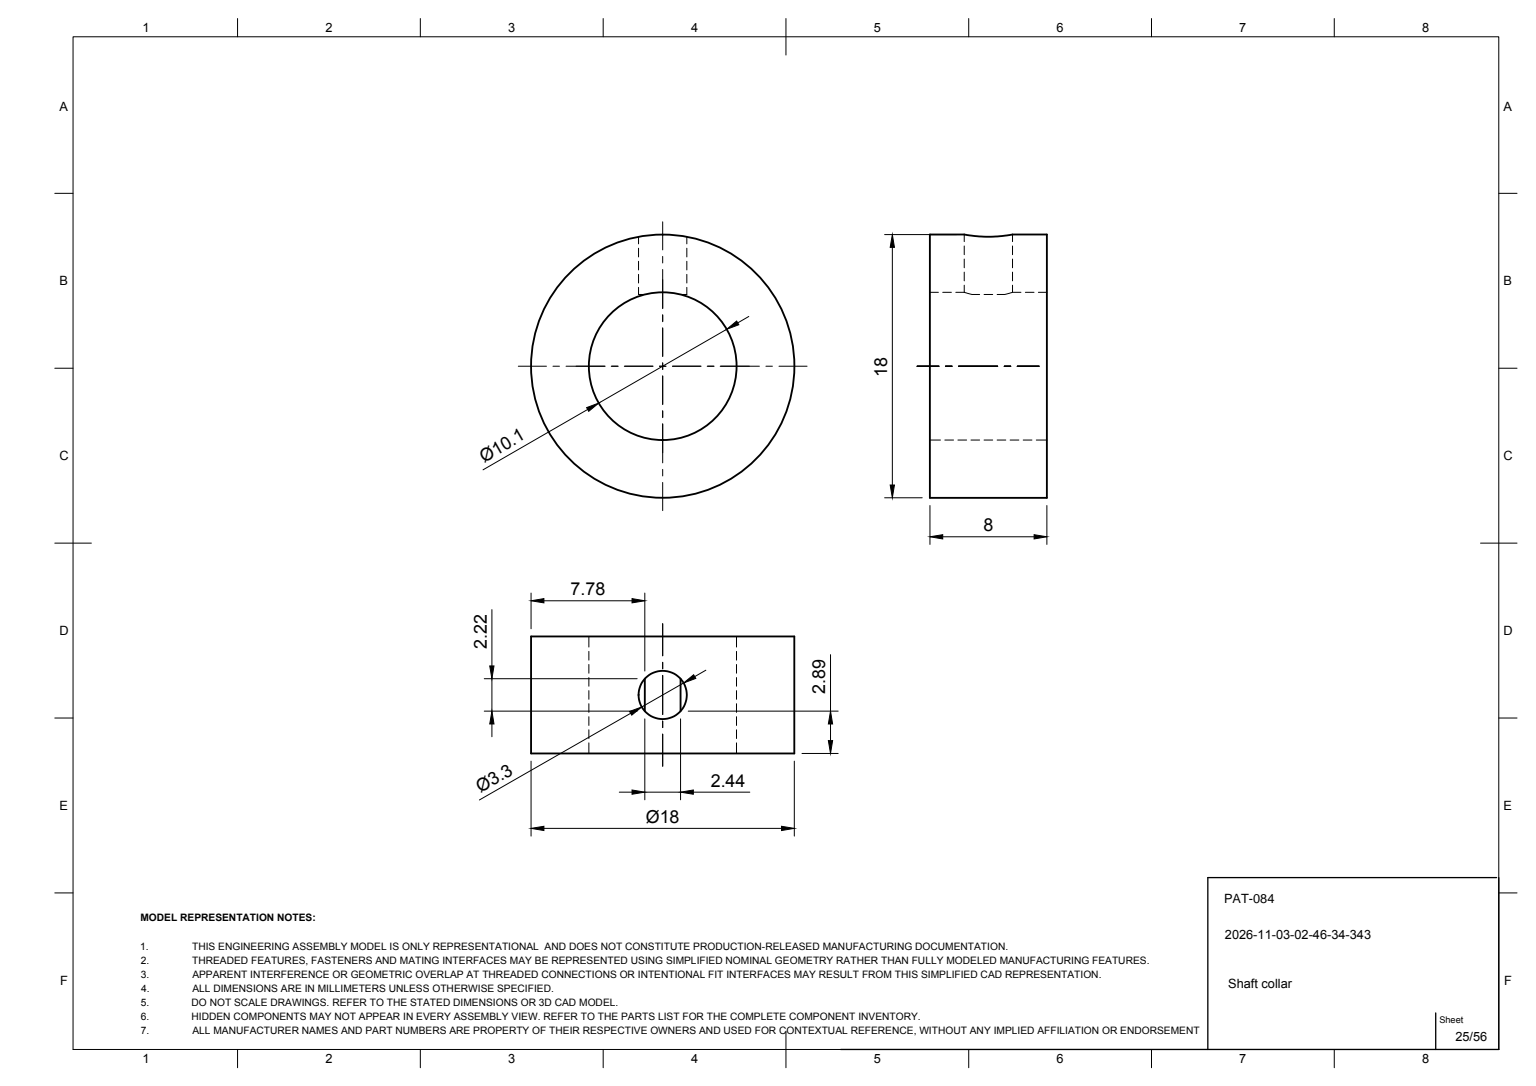
ISO-10303-21;
HEADER;
/* Generated by software containing ST-Developer
 * from STEP Tools, Inc. (www.steptools.com) 
 */

FILE_DESCRIPTION(
/* description */ ('Quick-return (Whitworth) mechanism'),
/* implementation_level */ '2;1');

FILE_NAME(
/* name */ 'Shaft collar.step',
/* time_stamp */ '2026-10-28T03:25:57-07:00',
/* author */ (''),
/* organization */ (''),
/* preprocessor_version */ 'ST-DEVELOPER v20.2',
/* originating_system */ 'Autodesk Translation Framework v15.17.0.0',
/* authorisation */ '');

FILE_SCHEMA (('AUTOMOTIVE_DESIGN { 1 0 10303 214 3 1 1 }'));
ENDSEC;

DATA;
#10=MECHANICAL_DESIGN_GEOMETRIC_PRESENTATION_REPRESENTATION('',(#514),#14878);
#392=B_SPLINE_CURVE_WITH_KNOTS('',3,(#13493,#13494,#13495,#13496,#13497,
#13498,#13499,#13500,#13501,#13502,#13503,#13504,#13505,#13506),
 .UNSPECIFIED.,.F.,.F.,(4,2,2,2,2,2,4),(0.618551524396291,0.626563103102765,
0.689203386094988,0.751843669087211,0.814483952079434,0.877124235071657,
0.88513581377813),.UNSPECIFIED.);
#393=B_SPLINE_CURVE_WITH_KNOTS('',3,(#13510,#13511,#13512,#13513,#13514,
#13515,#13516,#13517),.UNSPECIFIED.,.F.,.F.,(4,2,2,4),(0.250614556362404,
0.313254839354627,0.37589512234685,0.383906701053323),.UNSPECIFIED.);
#394=B_SPLINE_CURVE_WITH_KNOTS('',3,(#13521,#13522,#13523,#13524,#13525,
#13526,#13527,#13528,#13529,#13530,#13531,#13532,#13533,#13534,#13535,#13536,
#13537,#13538,#13539,#13540,#13541,#13542,#13543,#13544,#13545,#13546),
 .UNSPECIFIED.,.F.,.F.,(4,2,2,2,2,2,2,2,2,2,2,2,4),(0.,0.0623062782223143,
0.124612556444629,0.186916384615149,0.249220212785669,0.31152404095619,
0.37382786912671,0.436134147349024,0.498440425571339,0.560746703793653,
0.623052982015967,0.685356810186488,0.747660638357008),.UNSPECIFIED.);
#395=B_SPLINE_CURVE_WITH_KNOTS('',3,(#13547,#13548,#13549,#13550,#13551,
#13552,#13553,#13554,#13555,#13556),.UNSPECIFIED.,.F.,.F.,(4,2,2,2,4),(0.747660638357008,
0.809964466527529,0.872268294698049,0.934574572920363,0.996880851142677),
 .UNSPECIFIED.);
#396=B_SPLINE_CURVE_WITH_KNOTS('',3,(#13557,#13558,#13559,#13560,#13561,
#13562,#13563,#13564),.UNSPECIFIED.,.F.,.F.,(4,2,2,4),(0.117322411671485,
0.125333990377958,0.187974273370181,0.250614556362404),.UNSPECIFIED.);
#418=SHAPE_REPRESENTATION_RELATIONSHIP('SRR','None',#15088,#462);
#462=ADVANCED_BREP_SHAPE_REPRESENTATION('',(#566),#14845);
#514=STYLED_ITEM('',(#15406),#566);
#566=MANIFOLD_SOLID_BREP('Body1',#7868);
#711=FACE_BOUND('',#1863,.T.);
#712=FACE_BOUND('',#1865,.T.);
#713=FACE_BOUND('',#1867,.T.);
#714=FACE_BOUND('',#1869,.T.);
#886=PLANE('',#8896);
#887=PLANE('',#8900);
#888=PLANE('',#8907);
#889=PLANE('',#8908);
#1273=FACE_OUTER_BOUND('',#1859,.T.);
#1274=FACE_OUTER_BOUND('',#1860,.T.);
#1275=FACE_OUTER_BOUND('',#1861,.T.);
#1276=FACE_OUTER_BOUND('',#1862,.T.);
#1277=FACE_OUTER_BOUND('',#1864,.T.);
#1278=FACE_OUTER_BOUND('',#1866,.T.);
#1279=FACE_OUTER_BOUND('',#1868,.T.);
#1859=EDGE_LOOP('',(#6226,#6227));
#1860=EDGE_LOOP('',(#6228,#6229,#6230,#6231,#6232,#6233,#6234,#6235,#6236));
#1861=EDGE_LOOP('',(#6237,#6238));
#1862=EDGE_LOOP('',(#6239,#6240,#6241,#6242));
#1863=EDGE_LOOP('',(#6243,#6244,#6245,#6246,#6247));
#1864=EDGE_LOOP('',(#6248,#6249,#6250,#6251));
#1865=EDGE_LOOP('',(#6252,#6253));
#1866=EDGE_LOOP('',(#6254));
#1867=EDGE_LOOP('',(#6255));
#1868=EDGE_LOOP('',(#6256));
#1869=EDGE_LOOP('',(#6257));
#2366=LINE('',#13489,#2889);
#2367=LINE('',#13519,#2890);
#2368=LINE('',#13566,#2891);
#2369=LINE('',#13571,#2892);
#2370=LINE('',#13577,#2893);
#2889=VECTOR('',#10619,1.);
#2890=VECTOR('',#10626,0.165);
#2891=VECTOR('',#10629,1.);
#2892=VECTOR('',#10634,0.505);
#2893=VECTOR('',#10641,0.9);
#3476=CIRCLE('',#8897,0.165);
#3477=CIRCLE('',#8899,0.165);
#3478=CIRCLE('',#8902,0.505);
#3479=CIRCLE('',#8903,0.505);
#3480=CIRCLE('',#8905,0.9);
#3481=CIRCLE('',#8906,0.9);
#3963=VERTEX_POINT('',#13487);
#3964=VERTEX_POINT('',#13488);
#3965=VERTEX_POINT('',#13492);
#3966=VERTEX_POINT('',#13507);
#3967=VERTEX_POINT('',#13509);
#3968=VERTEX_POINT('',#13518);
#3969=VERTEX_POINT('',#13520);
#3970=VERTEX_POINT('',#13568);
#3971=VERTEX_POINT('',#13570);
#3972=VERTEX_POINT('',#13574);
#3973=VERTEX_POINT('',#13576);
#4770=EDGE_CURVE('',#3963,#3964,#2366,.T.);
#4771=EDGE_CURVE('',#3963,#3964,#3476,.T.);
#4772=EDGE_CURVE('',#3965,#3963,#392,.T.);
#4773=EDGE_CURVE('',#3966,#3965,#3477,.T.);
#4774=EDGE_CURVE('',#3967,#3966,#393,.T.);
#4775=EDGE_CURVE('',#3967,#3968,#2367,.T.);
#4776=EDGE_CURVE('',#3969,#3968,#394,.T.);
#4777=EDGE_CURVE('',#3968,#3969,#395,.T.);
#4778=EDGE_CURVE('',#3964,#3967,#396,.T.);
#4779=EDGE_CURVE('',#3966,#3965,#2368,.T.);
#4780=EDGE_CURVE('',#3970,#3970,#3478,.T.);
#4781=EDGE_CURVE('',#3970,#3971,#2369,.T.);
#4782=EDGE_CURVE('',#3971,#3971,#3479,.T.);
#4783=EDGE_CURVE('',#3972,#3972,#3480,.T.);
#4784=EDGE_CURVE('',#3972,#3973,#2370,.T.);
#4785=EDGE_CURVE('',#3973,#3973,#3481,.T.);
#6226=ORIENTED_EDGE('',*,*,#4770,.F.);
#6227=ORIENTED_EDGE('',*,*,#4771,.T.);
#6228=ORIENTED_EDGE('',*,*,#4772,.F.);
#6229=ORIENTED_EDGE('',*,*,#4773,.F.);
#6230=ORIENTED_EDGE('',*,*,#4774,.F.);
#6231=ORIENTED_EDGE('',*,*,#4775,.T.);
#6232=ORIENTED_EDGE('',*,*,#4776,.F.);
#6233=ORIENTED_EDGE('',*,*,#4777,.F.);
#6234=ORIENTED_EDGE('',*,*,#4775,.F.);
#6235=ORIENTED_EDGE('',*,*,#4778,.F.);
#6236=ORIENTED_EDGE('',*,*,#4771,.F.);
#6237=ORIENTED_EDGE('',*,*,#4779,.F.);
#6238=ORIENTED_EDGE('',*,*,#4773,.T.);
#6239=ORIENTED_EDGE('',*,*,#4780,.F.);
#6240=ORIENTED_EDGE('',*,*,#4781,.T.);
#6241=ORIENTED_EDGE('',*,*,#4782,.T.);
#6242=ORIENTED_EDGE('',*,*,#4781,.F.);
#6243=ORIENTED_EDGE('',*,*,#4778,.T.);
#6244=ORIENTED_EDGE('',*,*,#4774,.T.);
#6245=ORIENTED_EDGE('',*,*,#4779,.T.);
#6246=ORIENTED_EDGE('',*,*,#4772,.T.);
#6247=ORIENTED_EDGE('',*,*,#4770,.T.);
#6248=ORIENTED_EDGE('',*,*,#4783,.F.);
#6249=ORIENTED_EDGE('',*,*,#4784,.T.);
#6250=ORIENTED_EDGE('',*,*,#4785,.T.);
#6251=ORIENTED_EDGE('',*,*,#4784,.F.);
#6252=ORIENTED_EDGE('',*,*,#4776,.T.);
#6253=ORIENTED_EDGE('',*,*,#4777,.T.);
#6254=ORIENTED_EDGE('',*,*,#4783,.T.);
#6255=ORIENTED_EDGE('',*,*,#4780,.T.);
#6256=ORIENTED_EDGE('',*,*,#4785,.F.);
#6257=ORIENTED_EDGE('',*,*,#4782,.F.);
#7310=CYLINDRICAL_SURFACE('',#8898,0.165);
#7311=CYLINDRICAL_SURFACE('',#8901,0.505);
#7312=CYLINDRICAL_SURFACE('',#8904,0.9);
#7604=ADVANCED_FACE('',(#1273),#886,.T.);
#7605=ADVANCED_FACE('',(#1274),#7310,.F.);
#7606=ADVANCED_FACE('',(#1275),#887,.T.);
#7607=ADVANCED_FACE('',(#1276,#711),#7311,.F.);
#7608=ADVANCED_FACE('',(#1277,#712),#7312,.T.);
#7609=ADVANCED_FACE('',(#1278,#713),#888,.T.);
#7610=ADVANCED_FACE('',(#1279,#714),#889,.F.);
#7868=CLOSED_SHELL('',(#7604,#7605,#7606,#7607,#7608,#7609,#7610));
#8895=AXIS2_PLACEMENT_3D('',#13485,#10615,#10616);
#8896=AXIS2_PLACEMENT_3D('',#13486,#10617,#10618);
#8897=AXIS2_PLACEMENT_3D('',#13490,#10620,#10621);
#8898=AXIS2_PLACEMENT_3D('',#13491,#10622,#10623);
#8899=AXIS2_PLACEMENT_3D('',#13508,#10624,#10625);
#8900=AXIS2_PLACEMENT_3D('',#13565,#10627,#10628);
#8901=AXIS2_PLACEMENT_3D('',#13567,#10630,#10631);
#8902=AXIS2_PLACEMENT_3D('',#13569,#10632,#10633);
#8903=AXIS2_PLACEMENT_3D('',#13572,#10635,#10636);
#8904=AXIS2_PLACEMENT_3D('',#13573,#10637,#10638);
#8905=AXIS2_PLACEMENT_3D('',#13575,#10639,#10640);
#8906=AXIS2_PLACEMENT_3D('',#13578,#10642,#10643);
#8907=AXIS2_PLACEMENT_3D('',#13579,#10644,#10645);
#8908=AXIS2_PLACEMENT_3D('',#13580,#10646,#10647);
#10615=DIRECTION('axis',(0.,0.,1.));
#10616=DIRECTION('refdir',(1.,0.,0.));
#10617=DIRECTION('center_axis',(1.,0.,0.));
#10618=DIRECTION('ref_axis',(0.,0.,-1.));
#10619=DIRECTION('',(0.,0.,1.));
#10620=DIRECTION('center_axis',(1.,0.,0.));
#10621=DIRECTION('ref_axis',(0.,0.,-1.));
#10622=DIRECTION('center_axis',(1.,0.,0.));
#10623=DIRECTION('ref_axis',(0.,0.,-1.));
#10624=DIRECTION('center_axis',(1.,0.,0.));
#10625=DIRECTION('ref_axis',(0.,0.,-1.));
#10626=DIRECTION('',(1.,0.,0.));
#10627=DIRECTION('center_axis',(1.,0.,0.));
#10628=DIRECTION('ref_axis',(0.,0.,-1.));
#10629=DIRECTION('',(0.,0.,-1.));
#10630=DIRECTION('center_axis',(0.,0.,1.));
#10631=DIRECTION('ref_axis',(1.,0.,0.));
#10632=DIRECTION('center_axis',(0.,0.,-1.));
#10633=DIRECTION('ref_axis',(1.,0.,0.));
#10634=DIRECTION('',(0.,0.,-1.));
#10635=DIRECTION('center_axis',(0.,0.,-1.));
#10636=DIRECTION('ref_axis',(1.,0.,0.));
#10637=DIRECTION('center_axis',(0.,0.,1.));
#10638=DIRECTION('ref_axis',(1.,0.,0.));
#10639=DIRECTION('center_axis',(0.,0.,1.));
#10640=DIRECTION('ref_axis',(1.,0.,0.));
#10641=DIRECTION('',(0.,0.,-1.));
#10642=DIRECTION('center_axis',(0.,0.,1.));
#10643=DIRECTION('ref_axis',(1.,0.,0.));
#10644=DIRECTION('center_axis',(0.,0.,1.));
#10645=DIRECTION('ref_axis',(1.,0.,0.));
#10646=DIRECTION('center_axis',(0.,0.,1.));
#10647=DIRECTION('ref_axis',(1.,0.,0.));
#13485=CARTESIAN_POINT('',(0.,0.,0.));
#13486=CARTESIAN_POINT('Origin',(0.49,6.,1.4));
#13487=CARTESIAN_POINT('',(0.49,6.12216791722871,1.28909463493591));
#13488=CARTESIAN_POINT('',(0.49,6.12216791722871,1.51090536506409));
#13489=CARTESIAN_POINT('',(0.49,6.12216791722871,1.));
#13490=CARTESIAN_POINT('Origin',(0.49,6.,1.4));
#13491=CARTESIAN_POINT('Origin',(0.49,6.,1.4));
#13492=CARTESIAN_POINT('',(0.49,5.87783208277129,1.28909463493591));
#13493=CARTESIAN_POINT('Ctrl Pts',(0.49,5.87783208277129,1.28909463493591));
#13494=CARTESIAN_POINT('Ctrl Pts',(0.490448531679987,5.8796310863737,1.28711294069536));
#13495=CARTESIAN_POINT('Ctrl Pts',(0.490895245371684,5.88146510343477,1.28518965877367));
#13496=CARTESIAN_POINT('Ctrl Pts',(0.494795015531646,5.89788800698064,1.2687667552278));
#13497=CARTESIAN_POINT('Ctrl Pts',(0.498442514607594,5.91634028497757,1.25609154388858));
#13498=CARTESIAN_POINT('Ctrl Pts',(0.50357781976106,5.95695040395284,1.23920409039234));
#13499=CARTESIAN_POINT('Ctrl Pts',(0.505,5.97911990566926,1.235));
#13500=CARTESIAN_POINT('Ctrl Pts',(0.505,6.02088009433074,1.235));
#13501=CARTESIAN_POINT('Ctrl Pts',(0.50357781976106,6.04304959604716,1.23920409039234));
#13502=CARTESIAN_POINT('Ctrl Pts',(0.498442514607594,6.08365971502243,1.25609154388858));
#13503=CARTESIAN_POINT('Ctrl Pts',(0.494795015531646,6.10211199301936,1.2687667552278));
#13504=CARTESIAN_POINT('Ctrl Pts',(0.490895245371684,6.11853489656523,1.28518965877367));
#13505=CARTESIAN_POINT('Ctrl Pts',(0.490448531679987,6.1203689136263,1.28711294069536));
#13506=CARTESIAN_POINT('Ctrl Pts',(0.49,6.12216791722871,1.28909463493591));
#13507=CARTESIAN_POINT('',(0.49,5.87783208277129,1.51090536506409));
#13508=CARTESIAN_POINT('Origin',(0.49,6.,1.4));
#13509=CARTESIAN_POINT('',(0.505,6.,1.565));
#13510=CARTESIAN_POINT('Ctrl Pts',(0.505,6.,1.565));
#13511=CARTESIAN_POINT('Ctrl Pts',(0.505,5.97911990566926,1.565));
#13512=CARTESIAN_POINT('Ctrl Pts',(0.50357781976106,5.95695040395284,1.56079590960766));
#13513=CARTESIAN_POINT('Ctrl Pts',(0.498442514607594,5.91634028497757,1.54390845611142));
#13514=CARTESIAN_POINT('Ctrl Pts',(0.494795015531646,5.89788800698064,1.5312332447722));
#13515=CARTESIAN_POINT('Ctrl Pts',(0.490895245371684,5.88146510343477,1.51481034122633));
#13516=CARTESIAN_POINT('Ctrl Pts',(0.490448531679987,5.8796310863737,1.51288705930464));
#13517=CARTESIAN_POINT('Ctrl Pts',(0.49,5.87783208277129,1.51090536506409));
#13518=CARTESIAN_POINT('',(0.9,6.,1.565));
#13519=CARTESIAN_POINT('',(0.49,6.,1.565));
#13520=CARTESIAN_POINT('',(0.884745726183518,6.165,1.4));
#13521=CARTESIAN_POINT('Ctrl Pts',(0.884745726183518,6.165,1.4));
#13522=CARTESIAN_POINT('Ctrl Pts',(0.884745726183518,6.165,1.37923124059256));
#13523=CARTESIAN_POINT('Ctrl Pts',(0.885552759505264,6.16083971900758,1.35711110492666));
#13524=CARTESIAN_POINT('Ctrl Pts',(0.888448648150043,6.14398647021669,1.31647293736623));
#13525=CARTESIAN_POINT('Ctrl Pts',(0.890493604851638,6.13129599381419,1.29795075602263));
#13526=CARTESIAN_POINT('Ctrl Pts',(0.89431723432394,6.10204981900812,1.26870458121656));
#13527=CARTESIAN_POINT('Ctrl Pts',(0.896347088899543,6.08352739209068,1.25601365401642));
#13528=CARTESIAN_POINT('Ctrl Pts',(0.899208271860583,6.04288837609341,1.23916007816136));
#13529=CARTESIAN_POINT('Ctrl Pts',(0.9,6.02076794272351,1.235));
#13530=CARTESIAN_POINT('Ctrl Pts',(0.9,5.97923205727649,1.235));
#13531=CARTESIAN_POINT('Ctrl Pts',(0.899208271860583,5.95711162390659,1.23916007816136));
#13532=CARTESIAN_POINT('Ctrl Pts',(0.896347088899543,5.91647260790932,1.25601365401642));
#13533=CARTESIAN_POINT('Ctrl Pts',(0.89431723432394,5.89795018099188,1.26870458121656));
#13534=CARTESIAN_POINT('Ctrl Pts',(0.890493604851638,5.86870400618581,1.29795075602263));
#13535=CARTESIAN_POINT('Ctrl Pts',(0.888448648150043,5.85601352978331,1.31647293736623));
#13536=CARTESIAN_POINT('Ctrl Pts',(0.885552759505264,5.83916028099242,1.35711110492666));
#13537=CARTESIAN_POINT('Ctrl Pts',(0.884745726183518,5.835,1.37923124059256));
#13538=CARTESIAN_POINT('Ctrl Pts',(0.884745726183518,5.835,1.42076875940744));
#13539=CARTESIAN_POINT('Ctrl Pts',(0.885552759505264,5.83916028099242,1.44288889507334));
#13540=CARTESIAN_POINT('Ctrl Pts',(0.888448648150043,5.85601352978331,1.48352706263377));
#13541=CARTESIAN_POINT('Ctrl Pts',(0.890493604851638,5.86870400618581,1.50204924397737));
#13542=CARTESIAN_POINT('Ctrl Pts',(0.89431723432394,5.89795018099188,1.53129541878344));
#13543=CARTESIAN_POINT('Ctrl Pts',(0.896347088899543,5.91647260790932,1.54398634598358));
#13544=CARTESIAN_POINT('Ctrl Pts',(0.899208271860583,5.95711162390659,1.56083992183864));
#13545=CARTESIAN_POINT('Ctrl Pts',(0.9,5.97923205727649,1.565));
#13546=CARTESIAN_POINT('Ctrl Pts',(0.9,6.,1.565));
#13547=CARTESIAN_POINT('Ctrl Pts',(0.9,6.,1.565));
#13548=CARTESIAN_POINT('Ctrl Pts',(0.9,6.02076794272351,1.565));
#13549=CARTESIAN_POINT('Ctrl Pts',(0.899208271860583,6.04288837609341,1.56083992183864));
#13550=CARTESIAN_POINT('Ctrl Pts',(0.896347088899543,6.08352739209068,1.54398634598358));
#13551=CARTESIAN_POINT('Ctrl Pts',(0.89431723432394,6.10204981900812,1.53129541878344));
#13552=CARTESIAN_POINT('Ctrl Pts',(0.890493604851638,6.13129599381419,1.50204924397737));
#13553=CARTESIAN_POINT('Ctrl Pts',(0.888448648150043,6.14398647021669,1.48352706263377));
#13554=CARTESIAN_POINT('Ctrl Pts',(0.885552759505264,6.16083971900758,1.44288889507334));
#13555=CARTESIAN_POINT('Ctrl Pts',(0.884745726183518,6.165,1.42076875940744));
#13556=CARTESIAN_POINT('Ctrl Pts',(0.884745726183518,6.165,1.4));
#13557=CARTESIAN_POINT('Ctrl Pts',(0.49,6.12216791722871,1.51090536506409));
#13558=CARTESIAN_POINT('Ctrl Pts',(0.490448531679987,6.1203689136263,1.51288705930464));
#13559=CARTESIAN_POINT('Ctrl Pts',(0.490895245371684,6.11853489656523,1.51481034122633));
#13560=CARTESIAN_POINT('Ctrl Pts',(0.494795015531646,6.10211199301936,1.5312332447722));
#13561=CARTESIAN_POINT('Ctrl Pts',(0.498442514607594,6.08365971502243,1.54390845611142));
#13562=CARTESIAN_POINT('Ctrl Pts',(0.50357781976106,6.04304959604716,1.56079590960766));
#13563=CARTESIAN_POINT('Ctrl Pts',(0.505,6.02088009433074,1.565));
#13564=CARTESIAN_POINT('Ctrl Pts',(0.505,6.,1.565));
#13565=CARTESIAN_POINT('Origin',(0.49,6.,1.4));
#13566=CARTESIAN_POINT('',(0.49,5.87783208277129,1.));
#13567=CARTESIAN_POINT('Origin',(0.,6.,1.));
#13568=CARTESIAN_POINT('',(-0.505,6.,1.8));
#13569=CARTESIAN_POINT('Origin',(0.,6.,1.8));
#13570=CARTESIAN_POINT('',(-0.505,6.,1.));
#13571=CARTESIAN_POINT('',(-0.505,6.,1.));
#13572=CARTESIAN_POINT('Origin',(0.,6.,1.));
#13573=CARTESIAN_POINT('Origin',(0.,6.,1.));
#13574=CARTESIAN_POINT('',(-0.9,6.,1.8));
#13575=CARTESIAN_POINT('Origin',(0.,6.,1.8));
#13576=CARTESIAN_POINT('',(-0.9,6.,1.));
#13577=CARTESIAN_POINT('',(-0.9,6.,1.));
#13578=CARTESIAN_POINT('Origin',(0.,6.,1.));
#13579=CARTESIAN_POINT('Origin',(0.,6.,1.8));
#13580=CARTESIAN_POINT('Origin',(0.,6.,1.));
#14791=UNCERTAINTY_MEASURE_WITH_UNIT(LENGTH_MEASURE(0.001),#14879,
'DISTANCE_ACCURACY_VALUE',
'Maximum model space distance between geometric entities at asserted c
onnectivities');
#14824=UNCERTAINTY_MEASURE_WITH_UNIT(LENGTH_MEASURE(0.001),#14879,
'DISTANCE_ACCURACY_VALUE',
'Maximum model space distance between geometric entities at asserted c
onnectivities');
#14845=(
GEOMETRIC_REPRESENTATION_CONTEXT(3)
GLOBAL_UNCERTAINTY_ASSIGNED_CONTEXT((#14791))
GLOBAL_UNIT_ASSIGNED_CONTEXT((#14879,#14881,#14882))
REPRESENTATION_CONTEXT('','3D')
);
#14878=(
GEOMETRIC_REPRESENTATION_CONTEXT(3)
GLOBAL_UNCERTAINTY_ASSIGNED_CONTEXT((#14824))
GLOBAL_UNIT_ASSIGNED_CONTEXT((#14879,#14881,#14882))
REPRESENTATION_CONTEXT('','3D')
);
#14879=(
LENGTH_UNIT()
NAMED_UNIT(*)
SI_UNIT(.CENTI.,.METRE.)
);
#14881=(
NAMED_UNIT(*)
PLANE_ANGLE_UNIT()
SI_UNIT($,.RADIAN.)
);
#14882=(
NAMED_UNIT(*)
SI_UNIT($,.STERADIAN.)
SOLID_ANGLE_UNIT()
);
#14903=SHAPE_DEFINITION_REPRESENTATION(#14961,#15088);
#14961=PRODUCT_DEFINITION_SHAPE('',$,#15142);
#15088=SHAPE_REPRESENTATION('',(#8895),#14845);
#15121=PRODUCT_DEFINITION_CONTEXT('part definition',#15282,'design');
#15142=PRODUCT_DEFINITION('Shaft collar','Shaft collar',#15195,#15121);
#15195=PRODUCT_DEFINITION_FORMATION('',$,#15304);
#15282=APPLICATION_CONTEXT(
'Core Data for Automotive Mechanical Design Process');
#15283=PRODUCT_CONTEXT('part definition',#15282,'mechanical');
#15304=PRODUCT('Shaft collar','Shaft collar','Shaft collar',(#15283));
#15400=COLOUR_RGB('Grey',0.48,0.52,0.57);
#15401=FILL_AREA_STYLE_COLOUR('',#15400);
#15402=FILL_AREA_STYLE('',(#15401));
#15403=SURFACE_STYLE_FILL_AREA(#15402);
#15404=SURFACE_SIDE_STYLE('',(#15403));
#15405=SURFACE_STYLE_USAGE(.BOTH.,#15404);
#15406=PRESENTATION_STYLE_ASSIGNMENT((#15405));
ENDSEC;
END-ISO-10303-21;
